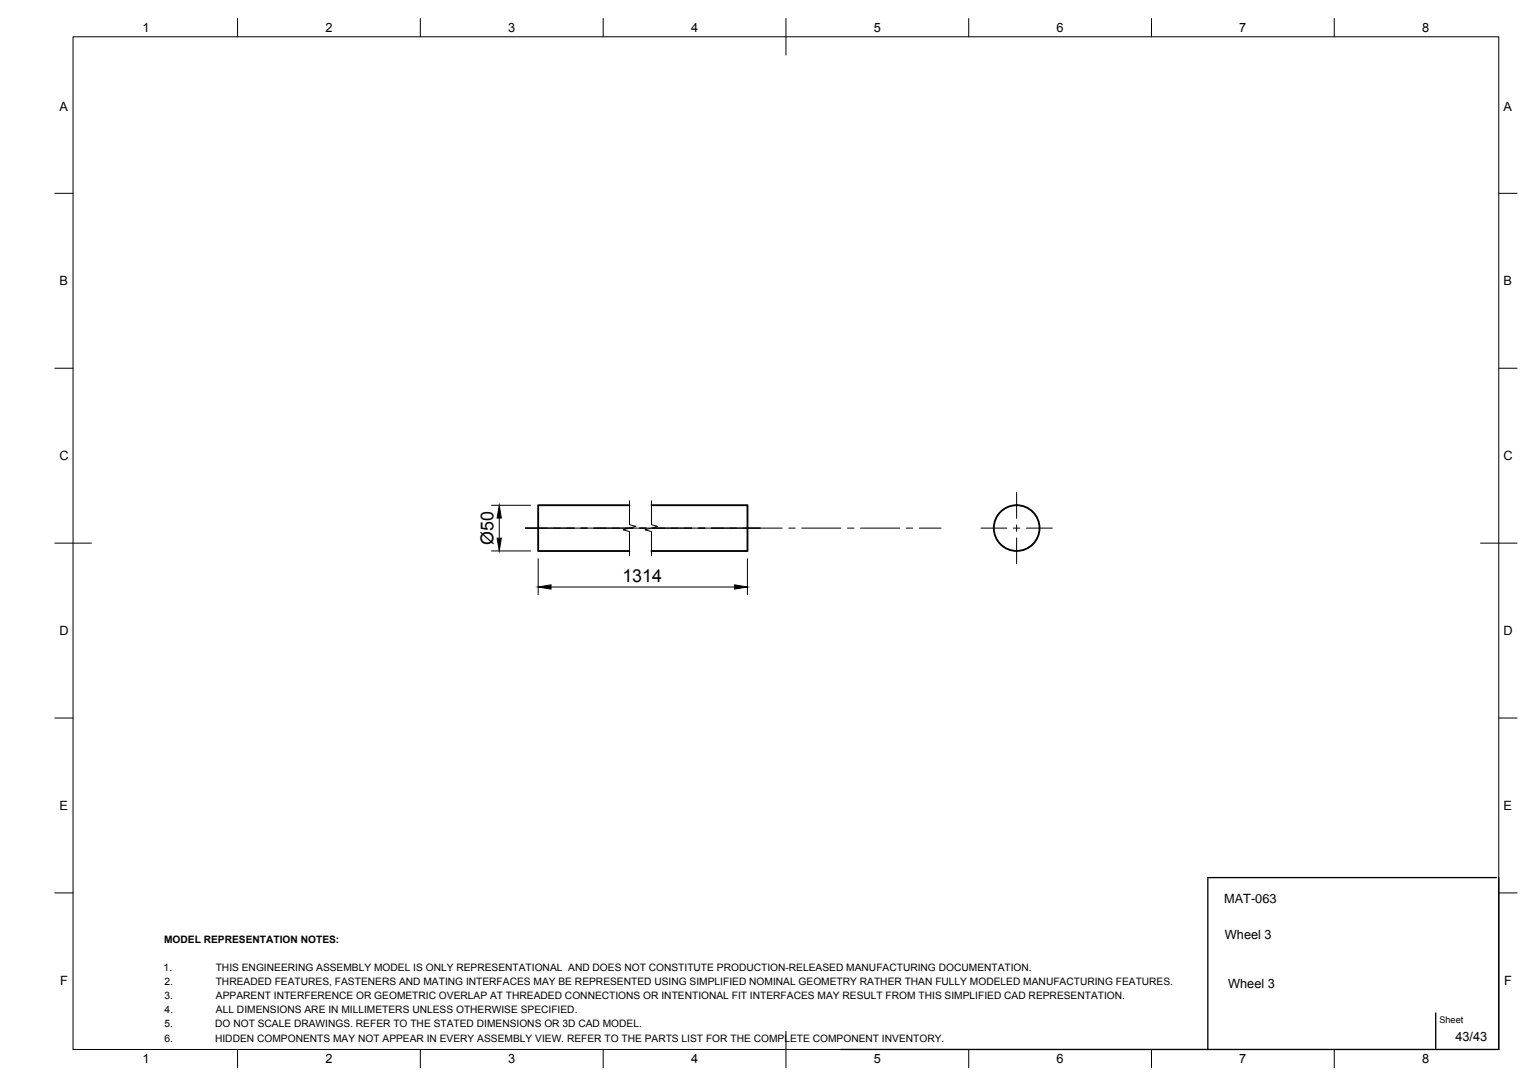
ISO-10303-21;
HEADER;
/* Generated by software containing ST-Developer
 * from STEP Tools, Inc. (www.steptools.com) 
 */

FILE_DESCRIPTION(
/* description */ (''),
/* implementation_level */ '2;1');

FILE_NAME(
/* name */ 'Wheel 3.step',
/* time_stamp */ '2026-10-24T09:43:01-07:00',
/* author */ (''),
/* organization */ (''),
/* preprocessor_version */ 'ST-DEVELOPER v20.2',
/* originating_system */ 'Autodesk Translation Framework v15.15.0.0',
/* authorisation */ '');

FILE_SCHEMA (('AUTOMOTIVE_DESIGN { 1 0 10303 214 3 1 1 }'));
ENDSEC;

DATA;
#10=MECHANICAL_DESIGN_GEOMETRIC_PRESENTATION_REPRESENTATION('',(#305),#11112);
#239=SHAPE_REPRESENTATION_RELATIONSHIP('SRR','None',#11266,#272);
#272=ADVANCED_BREP_SHAPE_REPRESENTATION('',(#338),#11111);
#305=STYLED_ITEM('',(#11426),#338);
#338=MANIFOLD_SOLID_BREP('Wheel 3',#6042);
#663=PLANE('',#7239);
#664=PLANE('',#7240);
#1034=FACE_OUTER_BOUND('',#1555,.T.);
#1035=FACE_OUTER_BOUND('',#1556,.T.);
#1036=FACE_OUTER_BOUND('',#1557,.T.);
#1555=EDGE_LOOP('',(#5493,#5494,#5495,#5496));
#1556=EDGE_LOOP('',(#5497));
#1557=EDGE_LOOP('',(#5498));
#1916=LINE('',#11012,#2275);
#2275=VECTOR('',#9280,0.025);
#2680=CIRCLE('',#7237,0.025);
#2681=CIRCLE('',#7238,0.025);
#3178=VERTEX_POINT('',#11009);
#3179=VERTEX_POINT('',#11011);
#3950=EDGE_CURVE('',#3178,#3178,#2680,.F.);
#3951=EDGE_CURVE('',#3178,#3179,#1916,.T.);
#3952=EDGE_CURVE('',#3179,#3179,#2681,.T.);
#5493=ORIENTED_EDGE('',*,*,#3950,.T.);
#5494=ORIENTED_EDGE('',*,*,#3951,.T.);
#5495=ORIENTED_EDGE('',*,*,#3952,.T.);
#5496=ORIENTED_EDGE('',*,*,#3951,.F.);
#5497=ORIENTED_EDGE('',*,*,#3952,.F.);
#5498=ORIENTED_EDGE('',*,*,#3950,.F.);
#5645=CYLINDRICAL_SURFACE('',#7236,0.025);
#6007=ADVANCED_FACE('',(#1034),#5645,.T.);
#6008=ADVANCED_FACE('',(#1035),#663,.T.);
#6009=ADVANCED_FACE('',(#1036),#664,.F.);
#6042=CLOSED_SHELL('',(#6007,#6008,#6009));
#7235=AXIS2_PLACEMENT_3D('',#11007,#9274,#9275);
#7236=AXIS2_PLACEMENT_3D('',#11008,#9276,#9277);
#7237=AXIS2_PLACEMENT_3D('',#11010,#9278,#9279);
#7238=AXIS2_PLACEMENT_3D('',#11013,#9281,#9282);
#7239=AXIS2_PLACEMENT_3D('',#11014,#9283,#9284);
#7240=AXIS2_PLACEMENT_3D('',#11015,#9285,#9286);
#9274=DIRECTION('axis',(0.,0.,1.));
#9275=DIRECTION('refdir',(1.,0.,0.));
#9276=DIRECTION('center_axis',(-1.,0.,0.));
#9277=DIRECTION('ref_axis',(0.,0.,1.));
#9278=DIRECTION('center_axis',(-1.,0.,0.));
#9279=DIRECTION('ref_axis',(0.,0.,1.));
#9280=DIRECTION('',(1.,0.,0.));
#9281=DIRECTION('center_axis',(-1.,0.,0.));
#9282=DIRECTION('ref_axis',(0.,0.,1.));
#9283=DIRECTION('center_axis',(1.,-4.74223835053899E-16,3.88578058810774E-16));
#9284=DIRECTION('ref_axis',(4.74223835053899E-16,1.,-6.83343688678077E-48));
#9285=DIRECTION('center_axis',(1.,4.74223835053899E-16,-3.88578058810774E-16));
#9286=DIRECTION('ref_axis',(-4.74223835053899E-16,1.,-6.83343688678077E-48));
#11007=CARTESIAN_POINT('',(0.,0.,0.));
#11008=CARTESIAN_POINT('Origin',(0.657,-0.386547301,0.));
#11009=CARTESIAN_POINT('',(-0.657,-0.386547301,-0.025));
#11010=CARTESIAN_POINT('Origin',(-0.657,-0.386547301,0.));
#11011=CARTESIAN_POINT('',(0.657,-0.386547301,-0.025));
#11012=CARTESIAN_POINT('',(0.657,-0.386547301,-0.025));
#11013=CARTESIAN_POINT('Origin',(0.657,-0.386547301,0.));
#11014=CARTESIAN_POINT('Origin',(0.657,-0.386547300999999,-2.61943244872498E-18));
#11015=CARTESIAN_POINT('Origin',(-0.657,-0.386547300999999,-2.61943244872498E-18));
#11072=UNCERTAINTY_MEASURE_WITH_UNIT(LENGTH_MEASURE(1.E-5),#11113,
'DISTANCE_ACCURACY_VALUE',
'Maximum model space distance between geometric entities at asserted c
onnectivities');
#11073=UNCERTAINTY_MEASURE_WITH_UNIT(LENGTH_MEASURE(1.E-5),#11113,
'DISTANCE_ACCURACY_VALUE',
'Maximum model space distance between geometric entities at asserted c
onnectivities');
#11111=(
GEOMETRIC_REPRESENTATION_CONTEXT(3)
GLOBAL_UNCERTAINTY_ASSIGNED_CONTEXT((#11072))
GLOBAL_UNIT_ASSIGNED_CONTEXT((#11113,#11114,#11115))
REPRESENTATION_CONTEXT('','3D')
);
#11112=(
GEOMETRIC_REPRESENTATION_CONTEXT(3)
GLOBAL_UNCERTAINTY_ASSIGNED_CONTEXT((#11073))
GLOBAL_UNIT_ASSIGNED_CONTEXT((#11113,#11114,#11115))
REPRESENTATION_CONTEXT('','3D')
);
#11113=(
LENGTH_UNIT()
NAMED_UNIT(*)
SI_UNIT($,.METRE.)
);
#11114=(
NAMED_UNIT(*)
PLANE_ANGLE_UNIT()
SI_UNIT($,.RADIAN.)
);
#11115=(
NAMED_UNIT(*)
SI_UNIT($,.STERADIAN.)
SOLID_ANGLE_UNIT()
);
#11153=SHAPE_DEFINITION_REPRESENTATION(#11209,#11266);
#11209=PRODUCT_DEFINITION_SHAPE('',$,#11305);
#11266=SHAPE_REPRESENTATION('',(#7235),#11111);
#11267=PRODUCT_DEFINITION_CONTEXT('part definition',#11383,'design');
#11305=PRODUCT_DEFINITION('Wheel 3','Wheel 3',#11343,#11267);
#11343=PRODUCT_DEFINITION_FORMATION('',$,#11422);
#11383=APPLICATION_CONTEXT(
'Core Data for Automotive Mechanical Design Process');
#11384=PRODUCT_CONTEXT('part definition',#11383,'mechanical');
#11422=PRODUCT('Wheel 3','Wheel 3','wheel__ DE     9829',(#11384));
#11426=PRESENTATION_STYLE_ASSIGNMENT((#11430));
#11430=SURFACE_STYLE_USAGE(.BOTH.,#11434);
#11434=SURFACE_SIDE_STYLE('',(#11438));
#11438=SURFACE_STYLE_FILL_AREA(#11442);
#11442=FILL_AREA_STYLE('Opaque(202,209,238)',(#11446));
#11446=FILL_AREA_STYLE_COLOUR('Opaque(202,209,238)',#11450);
#11450=COLOUR_RGB('Opaque(202,209,238)',0.792156862745098,0.819607843137255,
0.933333333333333);
ENDSEC;
END-ISO-10303-21;
